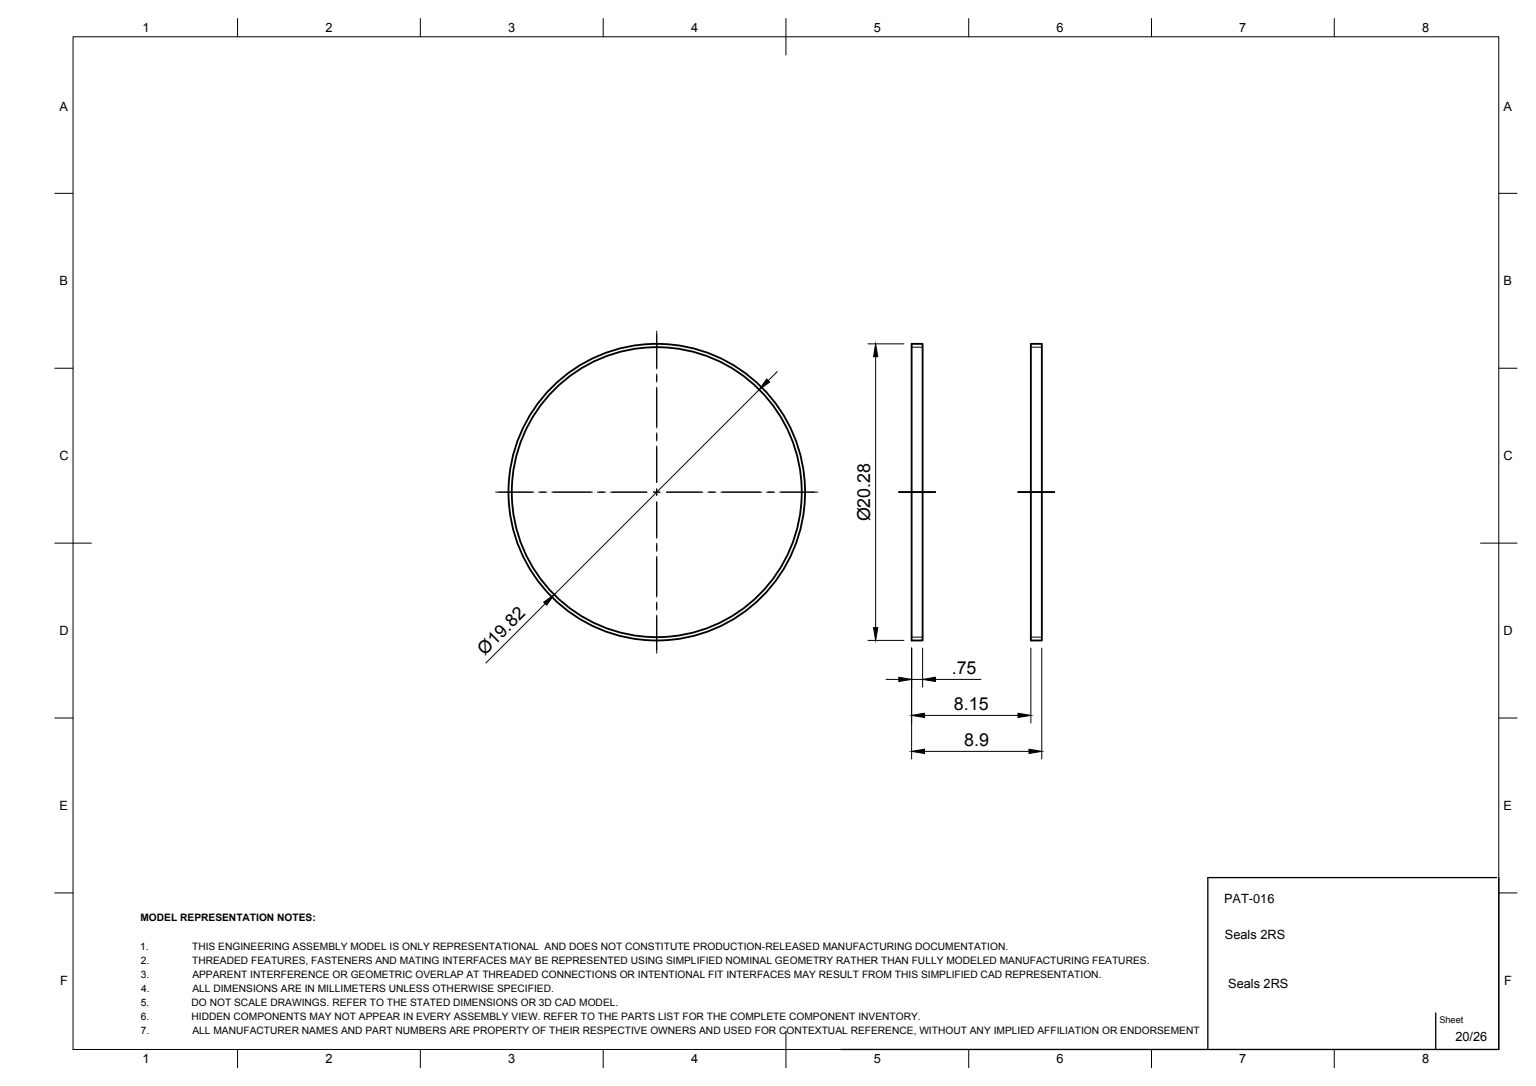
ISO-10303-21;
HEADER;
/* Generated by software containing ST-Developer
 * from STEP Tools, Inc. (www.steptools.com) 
 */

FILE_DESCRIPTION(
/* description */ ('Bracket-mounted idler roller'),
/* implementation_level */ '2;1');

FILE_NAME(
/* name */ 'Seals 2RS.step',
/* time_stamp */ '2026-10-28T03:26:42-07:00',
/* author */ (''),
/* organization */ (''),
/* preprocessor_version */ 'ST-DEVELOPER v20.2',
/* originating_system */ 'Autodesk Translation Framework v15.17.0.0',
/* authorisation */ '');

FILE_SCHEMA (('AUTOMOTIVE_DESIGN { 1 0 10303 214 3 1 1 }'));
ENDSEC;

DATA;
#10=MECHANICAL_DESIGN_GEOMETRIC_PRESENTATION_REPRESENTATION('',(#302,#303),#6241);
#253=SHAPE_REPRESENTATION_RELATIONSHIP('SRR','None',#6358,#274);
#274=ADVANCED_BREP_SHAPE_REPRESENTATION('',(#330,#331),#6234);
#302=STYLED_ITEM('',(#6538),#330);
#303=STYLED_ITEM('',(#6538),#331);
#330=MANIFOLD_SOLID_BREP('Body1',#3205);
#331=MANIFOLD_SOLID_BREP('Body2',#3206);
#378=FACE_BOUND('',#884,.T.);
#379=FACE_BOUND('',#887,.T.);
#380=FACE_BOUND('',#890,.T.);
#381=FACE_BOUND('',#893,.T.);
#491=PLANE('',#3719);
#492=PLANE('',#3724);
#493=PLANE('',#3727);
#494=PLANE('',#3732);
#650=FACE_OUTER_BOUND('',#883,.T.);
#651=FACE_OUTER_BOUND('',#885,.T.);
#652=FACE_OUTER_BOUND('',#886,.T.);
#653=FACE_OUTER_BOUND('',#888,.T.);
#654=FACE_OUTER_BOUND('',#889,.T.);
#655=FACE_OUTER_BOUND('',#891,.T.);
#656=FACE_OUTER_BOUND('',#892,.T.);
#657=FACE_OUTER_BOUND('',#894,.T.);
#883=EDGE_LOOP('',(#2708));
#884=EDGE_LOOP('',(#2709));
#885=EDGE_LOOP('',(#2710,#2711,#2712,#2713));
#886=EDGE_LOOP('',(#2714));
#887=EDGE_LOOP('',(#2715));
#888=EDGE_LOOP('',(#2716,#2717,#2718,#2719));
#889=EDGE_LOOP('',(#2720));
#890=EDGE_LOOP('',(#2721));
#891=EDGE_LOOP('',(#2722,#2723,#2724,#2725));
#892=EDGE_LOOP('',(#2726));
#893=EDGE_LOOP('',(#2727));
#894=EDGE_LOOP('',(#2728,#2729,#2730,#2731));
#1111=LINE('',#5909,#1293);
#1112=LINE('',#5914,#1294);
#1113=LINE('',#5923,#1295);
#1114=LINE('',#5928,#1296);
#1293=VECTOR('',#4576,1.013815);
#1294=VECTOR('',#4583,0.991185);
#1295=VECTOR('',#4594,1.013815);
#1296=VECTOR('',#4601,0.991185);
#1464=CIRCLE('',#3720,1.013815);
#1465=CIRCLE('',#3721,0.991185);
#1466=CIRCLE('',#3723,1.013815);
#1467=CIRCLE('',#3725,0.991185);
#1468=CIRCLE('',#3728,1.013815);
#1469=CIRCLE('',#3729,0.991185);
#1470=CIRCLE('',#3731,1.013815);
#1471=CIRCLE('',#3733,0.991185);
#1713=VERTEX_POINT('',#5902);
#1714=VERTEX_POINT('',#5904);
#1715=VERTEX_POINT('',#5907);
#1716=VERTEX_POINT('',#5911);
#1717=VERTEX_POINT('',#5916);
#1718=VERTEX_POINT('',#5918);
#1719=VERTEX_POINT('',#5921);
#1720=VERTEX_POINT('',#5925);
#2056=EDGE_CURVE('',#1713,#1713,#1464,.T.);
#2057=EDGE_CURVE('',#1714,#1714,#1465,.T.);
#2058=EDGE_CURVE('',#1715,#1715,#1466,.T.);
#2059=EDGE_CURVE('',#1715,#1713,#1111,.T.);
#2060=EDGE_CURVE('',#1716,#1716,#1467,.T.);
#2061=EDGE_CURVE('',#1716,#1714,#1112,.T.);
#2062=EDGE_CURVE('',#1717,#1717,#1468,.T.);
#2063=EDGE_CURVE('',#1718,#1718,#1469,.T.);
#2064=EDGE_CURVE('',#1719,#1719,#1470,.T.);
#2065=EDGE_CURVE('',#1719,#1717,#1113,.T.);
#2066=EDGE_CURVE('',#1720,#1720,#1471,.T.);
#2067=EDGE_CURVE('',#1720,#1718,#1114,.T.);
#2708=ORIENTED_EDGE('',*,*,#2056,.F.);
#2709=ORIENTED_EDGE('',*,*,#2057,.T.);
#2710=ORIENTED_EDGE('',*,*,#2058,.F.);
#2711=ORIENTED_EDGE('',*,*,#2059,.T.);
#2712=ORIENTED_EDGE('',*,*,#2056,.T.);
#2713=ORIENTED_EDGE('',*,*,#2059,.F.);
#2714=ORIENTED_EDGE('',*,*,#2058,.T.);
#2715=ORIENTED_EDGE('',*,*,#2060,.F.);
#2716=ORIENTED_EDGE('',*,*,#2060,.T.);
#2717=ORIENTED_EDGE('',*,*,#2061,.T.);
#2718=ORIENTED_EDGE('',*,*,#2057,.F.);
#2719=ORIENTED_EDGE('',*,*,#2061,.F.);
#2720=ORIENTED_EDGE('',*,*,#2062,.F.);
#2721=ORIENTED_EDGE('',*,*,#2063,.T.);
#2722=ORIENTED_EDGE('',*,*,#2064,.F.);
#2723=ORIENTED_EDGE('',*,*,#2065,.T.);
#2724=ORIENTED_EDGE('',*,*,#2062,.T.);
#2725=ORIENTED_EDGE('',*,*,#2065,.F.);
#2726=ORIENTED_EDGE('',*,*,#2064,.T.);
#2727=ORIENTED_EDGE('',*,*,#2066,.F.);
#2728=ORIENTED_EDGE('',*,*,#2066,.T.);
#2729=ORIENTED_EDGE('',*,*,#2067,.T.);
#2730=ORIENTED_EDGE('',*,*,#2063,.F.);
#2731=ORIENTED_EDGE('',*,*,#2067,.F.);
#2963=CYLINDRICAL_SURFACE('',#3722,1.013815);
#2964=CYLINDRICAL_SURFACE('',#3726,0.991185);
#2965=CYLINDRICAL_SURFACE('',#3730,1.013815);
#2966=CYLINDRICAL_SURFACE('',#3734,0.991185);
#3125=ADVANCED_FACE('',(#650,#378),#491,.T.);
#3126=ADVANCED_FACE('',(#651),#2963,.T.);
#3127=ADVANCED_FACE('',(#652,#379),#492,.T.);
#3128=ADVANCED_FACE('',(#653),#2964,.F.);
#3129=ADVANCED_FACE('',(#654,#380),#493,.T.);
#3130=ADVANCED_FACE('',(#655),#2965,.T.);
#3131=ADVANCED_FACE('',(#656,#381),#494,.T.);
#3132=ADVANCED_FACE('',(#657),#2966,.F.);
#3205=CLOSED_SHELL('',(#3125,#3126,#3127,#3128));
#3206=CLOSED_SHELL('',(#3129,#3130,#3131,#3132));
#3718=AXIS2_PLACEMENT_3D('',#5900,#4564,#4565);
#3719=AXIS2_PLACEMENT_3D('',#5901,#4566,#4567);
#3720=AXIS2_PLACEMENT_3D('',#5903,#4568,#4569);
#3721=AXIS2_PLACEMENT_3D('',#5905,#4570,#4571);
#3722=AXIS2_PLACEMENT_3D('',#5906,#4572,#4573);
#3723=AXIS2_PLACEMENT_3D('',#5908,#4574,#4575);
#3724=AXIS2_PLACEMENT_3D('',#5910,#4577,#4578);
#3725=AXIS2_PLACEMENT_3D('',#5912,#4579,#4580);
#3726=AXIS2_PLACEMENT_3D('',#5913,#4581,#4582);
#3727=AXIS2_PLACEMENT_3D('',#5915,#4584,#4585);
#3728=AXIS2_PLACEMENT_3D('',#5917,#4586,#4587);
#3729=AXIS2_PLACEMENT_3D('',#5919,#4588,#4589);
#3730=AXIS2_PLACEMENT_3D('',#5920,#4590,#4591);
#3731=AXIS2_PLACEMENT_3D('',#5922,#4592,#4593);
#3732=AXIS2_PLACEMENT_3D('',#5924,#4595,#4596);
#3733=AXIS2_PLACEMENT_3D('',#5926,#4597,#4598);
#3734=AXIS2_PLACEMENT_3D('',#5927,#4599,#4600);
#4564=DIRECTION('axis',(0.,0.,1.));
#4565=DIRECTION('refdir',(1.,0.,0.));
#4566=DIRECTION('center_axis',(0.,1.,0.));
#4567=DIRECTION('ref_axis',(0.,0.,1.));
#4568=DIRECTION('center_axis',(0.,-1.,0.));
#4569=DIRECTION('ref_axis',(1.,0.,0.));
#4570=DIRECTION('center_axis',(0.,-1.,0.));
#4571=DIRECTION('ref_axis',(1.,0.,0.));
#4572=DIRECTION('center_axis',(0.,-1.,0.));
#4573=DIRECTION('ref_axis',(1.,0.,0.));
#4574=DIRECTION('center_axis',(0.,-1.,0.));
#4575=DIRECTION('ref_axis',(1.,0.,0.));
#4576=DIRECTION('',(0.,1.,0.));
#4577=DIRECTION('center_axis',(0.,-1.,0.));
#4578=DIRECTION('ref_axis',(0.,0.,-1.));
#4579=DIRECTION('center_axis',(0.,-1.,0.));
#4580=DIRECTION('ref_axis',(1.,0.,0.));
#4581=DIRECTION('center_axis',(0.,-1.,0.));
#4582=DIRECTION('ref_axis',(1.,0.,0.));
#4583=DIRECTION('',(0.,1.,0.));
#4584=DIRECTION('center_axis',(0.,1.,0.));
#4585=DIRECTION('ref_axis',(0.,0.,1.));
#4586=DIRECTION('center_axis',(0.,-1.,0.));
#4587=DIRECTION('ref_axis',(1.,0.,0.));
#4588=DIRECTION('center_axis',(0.,-1.,0.));
#4589=DIRECTION('ref_axis',(1.,0.,0.));
#4590=DIRECTION('center_axis',(0.,-1.,0.));
#4591=DIRECTION('ref_axis',(1.,0.,0.));
#4592=DIRECTION('center_axis',(0.,-1.,0.));
#4593=DIRECTION('ref_axis',(1.,0.,0.));
#4594=DIRECTION('',(0.,1.,0.));
#4595=DIRECTION('center_axis',(0.,-1.,0.));
#4596=DIRECTION('ref_axis',(0.,0.,-1.));
#4597=DIRECTION('center_axis',(0.,-1.,0.));
#4598=DIRECTION('ref_axis',(1.,0.,0.));
#4599=DIRECTION('center_axis',(0.,-1.,0.));
#4600=DIRECTION('ref_axis',(1.,0.,0.));
#4601=DIRECTION('',(0.,1.,0.));
#5900=CARTESIAN_POINT('',(0.,0.,0.));
#5901=CARTESIAN_POINT('Origin',(1.013815,0.445,0.));
#5902=CARTESIAN_POINT('',(-1.013815,0.445,-1.24156529467757E-16));
#5903=CARTESIAN_POINT('Origin',(0.,0.445,0.));
#5904=CARTESIAN_POINT('',(-0.991185,0.445,-1.21385153761287E-16));
#5905=CARTESIAN_POINT('Origin',(0.,0.445,0.));
#5906=CARTESIAN_POINT('Origin',(0.,0.4075,0.));
#5907=CARTESIAN_POINT('',(-1.013815,0.37,-1.24156529467757E-16));
#5908=CARTESIAN_POINT('Origin',(0.,0.37,0.));
#5909=CARTESIAN_POINT('',(-1.013815,0.4075,-1.24156529467757E-16));
#5910=CARTESIAN_POINT('Origin',(0.991185,0.37,0.));
#5911=CARTESIAN_POINT('',(-0.991185,0.37,-1.21385153761287E-16));
#5912=CARTESIAN_POINT('Origin',(0.,0.37,0.));
#5913=CARTESIAN_POINT('Origin',(0.,0.4075,0.));
#5914=CARTESIAN_POINT('',(-0.991185,0.4075,-1.21385153761287E-16));
#5915=CARTESIAN_POINT('Origin',(1.013815,-0.37,0.));
#5916=CARTESIAN_POINT('',(-1.013815,-0.37,-1.24156529467757E-16));
#5917=CARTESIAN_POINT('Origin',(0.,-0.37,0.));
#5918=CARTESIAN_POINT('',(-0.991185,-0.37,-1.21385153761287E-16));
#5919=CARTESIAN_POINT('Origin',(0.,-0.37,0.));
#5920=CARTESIAN_POINT('Origin',(0.,-0.4075,0.));
#5921=CARTESIAN_POINT('',(-1.013815,-0.445,-1.24156529467757E-16));
#5922=CARTESIAN_POINT('Origin',(0.,-0.445,0.));
#5923=CARTESIAN_POINT('',(-1.013815,-0.4075,-1.24156529467757E-16));
#5924=CARTESIAN_POINT('Origin',(0.991185,-0.445,0.));
#5925=CARTESIAN_POINT('',(-0.991185,-0.445,-1.21385153761287E-16));
#5926=CARTESIAN_POINT('Origin',(0.,-0.445,0.));
#5927=CARTESIAN_POINT('Origin',(0.,-0.4075,0.));
#5928=CARTESIAN_POINT('',(-0.991185,-0.4075,-1.21385153761287E-16));
#6208=UNCERTAINTY_MEASURE_WITH_UNIT(LENGTH_MEASURE(0.001),#6242,
'DISTANCE_ACCURACY_VALUE',
'Maximum model space distance between geometric entities at asserted c
onnectivities');
#6215=UNCERTAINTY_MEASURE_WITH_UNIT(LENGTH_MEASURE(0.001),#6242,
'DISTANCE_ACCURACY_VALUE',
'Maximum model space distance between geometric entities at asserted c
onnectivities');
#6234=(
GEOMETRIC_REPRESENTATION_CONTEXT(3)
GLOBAL_UNCERTAINTY_ASSIGNED_CONTEXT((#6208))
GLOBAL_UNIT_ASSIGNED_CONTEXT((#6242,#6244,#6245))
REPRESENTATION_CONTEXT('','3D')
);
#6241=(
GEOMETRIC_REPRESENTATION_CONTEXT(3)
GLOBAL_UNCERTAINTY_ASSIGNED_CONTEXT((#6215))
GLOBAL_UNIT_ASSIGNED_CONTEXT((#6242,#6244,#6245))
REPRESENTATION_CONTEXT('','3D')
);
#6242=(
LENGTH_UNIT()
NAMED_UNIT(*)
SI_UNIT(.CENTI.,.METRE.)
);
#6244=(
NAMED_UNIT(*)
PLANE_ANGLE_UNIT()
SI_UNIT($,.RADIAN.)
);
#6245=(
NAMED_UNIT(*)
SI_UNIT($,.STERADIAN.)
SOLID_ANGLE_UNIT()
);
#6264=SHAPE_DEFINITION_REPRESENTATION(#6289,#6358);
#6289=PRODUCT_DEFINITION_SHAPE('',$,#6384);
#6358=SHAPE_REPRESENTATION('',(#3718),#6234);
#6365=PRODUCT_DEFINITION_CONTEXT('part definition',#6442,'design');
#6384=PRODUCT_DEFINITION('Seals 2RS','Seals 2RS',#6409,#6365);
#6409=PRODUCT_DEFINITION_FORMATION('',$,#6462);
#6442=APPLICATION_CONTEXT(
'Core Data for Automotive Mechanical Design Process');
#6443=PRODUCT_CONTEXT('part definition',#6442,'mechanical');
#6462=PRODUCT('Seals 2RS','Seals 2RS','Seals 2RS',(#6443));
#6532=COLOUR_RGB('Grey',0.48,0.52,0.57);
#6533=FILL_AREA_STYLE_COLOUR('',#6532);
#6534=FILL_AREA_STYLE('',(#6533));
#6535=SURFACE_STYLE_FILL_AREA(#6534);
#6536=SURFACE_SIDE_STYLE('',(#6535));
#6537=SURFACE_STYLE_USAGE(.BOTH.,#6536);
#6538=PRESENTATION_STYLE_ASSIGNMENT((#6537));
ENDSEC;
END-ISO-10303-21;
